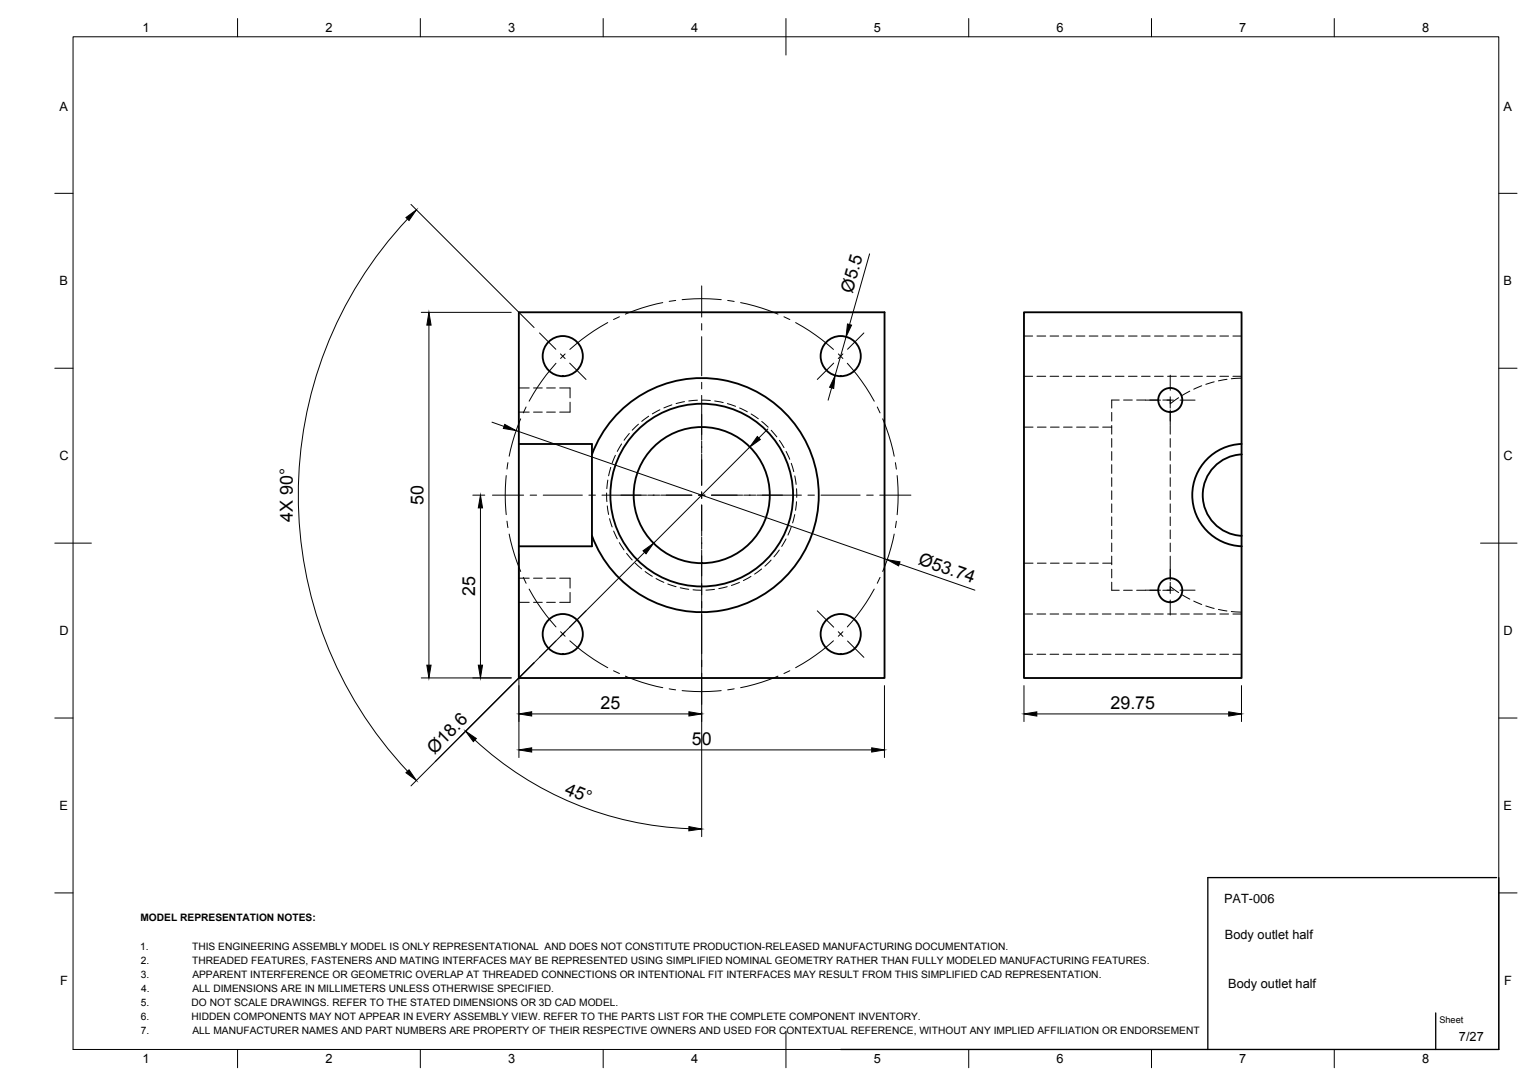
ISO-10303-21;
HEADER;
/* Generated by software containing ST-Developer
 * from STEP Tools, Inc. (www.steptools.com) 
 */

FILE_DESCRIPTION(
/* description */ ('Ball-type isolation valve (generic)'),
/* implementation_level */ '2;1');

FILE_NAME(
/* name */ 'Body outlet half.step',
/* time_stamp */ '2026-10-27T10:53:05-07:00',
/* author */ (''),
/* organization */ (''),
/* preprocessor_version */ 'ST-DEVELOPER v20.2',
/* originating_system */ 'Autodesk Translation Framework v15.17.0.0',
/* authorisation */ '');

FILE_SCHEMA (('AUTOMOTIVE_DESIGN { 1 0 10303 214 3 1 1 }'));
ENDSEC;

DATA;
#10=MECHANICAL_DESIGN_GEOMETRIC_PRESENTATION_REPRESENTATION('',(#279),#7425);
#227=SHAPE_REPRESENTATION_RELATIONSHIP('SRR','None',#7537,#253);
#253=ADVANCED_BREP_SHAPE_REPRESENTATION('',(#305),#7400);
#279=STYLED_ITEM('',(#7723),#305);
#305=MANIFOLD_SOLID_BREP('Body1',#4084);
#328=SPHERICAL_SURFACE('',#4490,1.6);
#348=FACE_BOUND('',#882,.T.);
#349=FACE_BOUND('',#883,.T.);
#350=FACE_BOUND('',#887,.T.);
#351=FACE_BOUND('',#889,.T.);
#352=FACE_BOUND('',#891,.T.);
#353=FACE_BOUND('',#893,.T.);
#354=FACE_BOUND('',#894,.T.);
#355=FACE_BOUND('',#895,.T.);
#356=FACE_BOUND('',#896,.T.);
#357=FACE_BOUND('',#897,.T.);
#358=FACE_BOUND('',#900,.T.);
#359=FACE_BOUND('',#901,.T.);
#360=FACE_BOUND('',#902,.T.);
#361=FACE_BOUND('',#903,.T.);
#432=PLANE('',#4458);
#433=PLANE('',#4462);
#434=PLANE('',#4478);
#435=PLANE('',#4480);
#436=PLANE('',#4487);
#437=PLANE('',#4488);
#438=PLANE('',#4492);
#439=PLANE('',#4493);
#440=PLANE('',#4494);
#441=PLANE('',#4495);
#442=PLANE('',#4496);
#605=FACE_OUTER_BOUND('',#871,.T.);
#606=FACE_OUTER_BOUND('',#872,.T.);
#607=FACE_OUTER_BOUND('',#873,.T.);
#608=FACE_OUTER_BOUND('',#874,.T.);
#609=FACE_OUTER_BOUND('',#875,.T.);
#610=FACE_OUTER_BOUND('',#876,.T.);
#611=FACE_OUTER_BOUND('',#877,.T.);
#612=FACE_OUTER_BOUND('',#878,.T.);
#613=FACE_OUTER_BOUND('',#879,.T.);
#614=FACE_OUTER_BOUND('',#880,.T.);
#615=FACE_OUTER_BOUND('',#881,.T.);
#616=FACE_OUTER_BOUND('',#884,.T.);
#617=FACE_OUTER_BOUND('',#885,.T.);
#618=FACE_OUTER_BOUND('',#886,.T.);
#619=FACE_OUTER_BOUND('',#888,.T.);
#620=FACE_OUTER_BOUND('',#890,.T.);
#621=FACE_OUTER_BOUND('',#892,.T.);
#622=FACE_OUTER_BOUND('',#898,.T.);
#623=FACE_OUTER_BOUND('',#899,.T.);
#624=FACE_OUTER_BOUND('',#904,.T.);
#625=FACE_OUTER_BOUND('',#905,.T.);
#871=EDGE_LOOP('',(#2881,#2882,#2883,#2884));
#872=EDGE_LOOP('',(#2885));
#873=EDGE_LOOP('',(#2886,#2887,#2888,#2889));
#874=EDGE_LOOP('',(#2890));
#875=EDGE_LOOP('',(#2891,#2892,#2893,#2894));
#876=EDGE_LOOP('',(#2895,#2896,#2897,#2898));
#877=EDGE_LOOP('',(#2899,#2900,#2901,#2902));
#878=EDGE_LOOP('',(#2903,#2904,#2905,#2906));
#879=EDGE_LOOP('',(#2907,#2908,#2909,#2910));
#880=EDGE_LOOP('',(#2911,#2912,#2913,#2914));
#881=EDGE_LOOP('',(#2915,#2916,#2917,#2918,#2919,#2920));
#882=EDGE_LOOP('',(#2921));
#883=EDGE_LOOP('',(#2922));
#884=EDGE_LOOP('',(#2923,#2924,#2925,#2926));
#885=EDGE_LOOP('',(#2927,#2928,#2929,#2930));
#886=EDGE_LOOP('',(#2931));
#887=EDGE_LOOP('',(#2932));
#888=EDGE_LOOP('',(#2933));
#889=EDGE_LOOP('',(#2934));
#890=EDGE_LOOP('',(#2935,#2936));
#891=EDGE_LOOP('',(#2937));
#892=EDGE_LOOP('',(#2938,#2939,#2940,#2941));
#893=EDGE_LOOP('',(#2942));
#894=EDGE_LOOP('',(#2943));
#895=EDGE_LOOP('',(#2944));
#896=EDGE_LOOP('',(#2945));
#897=EDGE_LOOP('',(#2946));
#898=EDGE_LOOP('',(#2947,#2948,#2949,#2950));
#899=EDGE_LOOP('',(#2951,#2952,#2953,#2954,#2955,#2956,#2957,#2958,#2959,
#2960));
#900=EDGE_LOOP('',(#2961));
#901=EDGE_LOOP('',(#2962));
#902=EDGE_LOOP('',(#2963));
#903=EDGE_LOOP('',(#2964));
#904=EDGE_LOOP('',(#2965,#2966,#2967,#2968));
#905=EDGE_LOOP('',(#2969,#2970,#2971,#2972));
#1192=LINE('',#6324,#1500);
#1193=LINE('',#6331,#1501);
#1194=LINE('',#6338,#1502);
#1195=LINE('',#6344,#1503);
#1196=LINE('',#6350,#1504);
#1197=LINE('',#6356,#1505);
#1198=LINE('',#6361,#1506);
#1199=LINE('',#6365,#1507);
#1200=LINE('',#6369,#1508);
#1201=LINE('',#6372,#1509);
#1202=LINE('',#6375,#1510);
#1203=LINE('',#6377,#1511);
#1204=LINE('',#6379,#1512);
#1205=LINE('',#6381,#1513);
#1206=LINE('',#6382,#1514);
#1207=LINE('',#6387,#1515);
#1208=LINE('',#6393,#1516);
#1209=LINE('',#6404,#1517);
#1210=LINE('',#6405,#1518);
#1211=LINE('',#6406,#1519);
#1212=LINE('',#6409,#1520);
#1213=LINE('',#6410,#1521);
#1214=LINE('',#6413,#1522);
#1215=LINE('',#6414,#1523);
#1216=LINE('',#6416,#1524);
#1500=VECTOR('',#5041,0.165);
#1501=VECTOR('',#5050,0.165);
#1502=VECTOR('',#5059,0.275);
#1503=VECTOR('',#5066,0.275);
#1504=VECTOR('',#5073,0.275);
#1505=VECTOR('',#5080,0.275);
#1506=VECTOR('',#5085,1.);
#1507=VECTOR('',#5088,1.);
#1508=VECTOR('',#5093,1.);
#1509=VECTOR('',#5096,1.);
#1510=VECTOR('',#5099,1.);
#1511=VECTOR('',#5100,1.);
#1512=VECTOR('',#5101,1.);
#1513=VECTOR('',#5102,1.);
#1514=VECTOR('',#5103,1.);
#1515=VECTOR('',#5108,0.93);
#1516=VECTOR('',#5115,1.3);
#1517=VECTOR('',#5130,1.);
#1518=VECTOR('',#5131,1.);
#1519=VECTOR('',#5132,1.);
#1520=VECTOR('',#5135,1.);
#1521=VECTOR('',#5136,1.);
#1522=VECTOR('',#5139,1.);
#1523=VECTOR('',#5140,1.);
#1524=VECTOR('',#5143,1.);
#1807=CIRCLE('',#4456,0.165);
#1808=CIRCLE('',#4457,0.165);
#1809=CIRCLE('',#4460,0.165);
#1810=CIRCLE('',#4461,0.165);
#1811=CIRCLE('',#4464,0.275);
#1812=CIRCLE('',#4465,0.275);
#1813=CIRCLE('',#4467,0.275);
#1814=CIRCLE('',#4468,0.275);
#1815=CIRCLE('',#4470,0.275);
#1816=CIRCLE('',#4471,0.275);
#1817=CIRCLE('',#4473,0.275);
#1818=CIRCLE('',#4474,0.275);
#1819=CIRCLE('',#4476,0.7);
#1820=CIRCLE('',#4477,0.7);
#1821=CIRCLE('',#4479,0.556776436283003);
#1822=CIRCLE('',#4482,0.93);
#1823=CIRCLE('',#4483,0.93);
#1824=CIRCLE('',#4485,1.3);
#1825=CIRCLE('',#4486,1.3);
#1826=CIRCLE('',#4489,1.24899959967968);
#1827=CIRCLE('',#4491,1.59980467557762);
#1992=VERTEX_POINT('',#6321);
#1993=VERTEX_POINT('',#6323);
#1994=VERTEX_POINT('',#6328);
#1995=VERTEX_POINT('',#6330);
#1996=VERTEX_POINT('',#6335);
#1997=VERTEX_POINT('',#6337);
#1998=VERTEX_POINT('',#6341);
#1999=VERTEX_POINT('',#6343);
#2000=VERTEX_POINT('',#6347);
#2001=VERTEX_POINT('',#6349);
#2002=VERTEX_POINT('',#6353);
#2003=VERTEX_POINT('',#6355);
#2004=VERTEX_POINT('',#6359);
#2005=VERTEX_POINT('',#6360);
#2006=VERTEX_POINT('',#6362);
#2007=VERTEX_POINT('',#6364);
#2008=VERTEX_POINT('',#6368);
#2009=VERTEX_POINT('',#6370);
#2010=VERTEX_POINT('',#6374);
#2011=VERTEX_POINT('',#6376);
#2012=VERTEX_POINT('',#6378);
#2013=VERTEX_POINT('',#6380);
#2014=VERTEX_POINT('',#6384);
#2015=VERTEX_POINT('',#6386);
#2016=VERTEX_POINT('',#6390);
#2017=VERTEX_POINT('',#6392);
#2018=VERTEX_POINT('',#6397);
#2019=VERTEX_POINT('',#6402);
#2020=VERTEX_POINT('',#6403);
#2021=VERTEX_POINT('',#6408);
#2022=VERTEX_POINT('',#6412);
#2333=EDGE_CURVE('',#1992,#1992,#1807,.T.);
#2334=EDGE_CURVE('',#1992,#1993,#1192,.T.);
#2335=EDGE_CURVE('',#1993,#1993,#1808,.T.);
#2336=EDGE_CURVE('',#1994,#1994,#1809,.T.);
#2337=EDGE_CURVE('',#1994,#1995,#1193,.T.);
#2338=EDGE_CURVE('',#1995,#1995,#1810,.T.);
#2339=EDGE_CURVE('',#1996,#1996,#1811,.T.);
#2340=EDGE_CURVE('',#1996,#1997,#1194,.T.);
#2341=EDGE_CURVE('',#1997,#1997,#1812,.T.);
#2342=EDGE_CURVE('',#1998,#1998,#1813,.T.);
#2343=EDGE_CURVE('',#1998,#1999,#1195,.T.);
#2344=EDGE_CURVE('',#1999,#1999,#1814,.T.);
#2345=EDGE_CURVE('',#2000,#2000,#1815,.T.);
#2346=EDGE_CURVE('',#2000,#2001,#1196,.T.);
#2347=EDGE_CURVE('',#2001,#2001,#1816,.T.);
#2348=EDGE_CURVE('',#2002,#2002,#1817,.T.);
#2349=EDGE_CURVE('',#2002,#2003,#1197,.T.);
#2350=EDGE_CURVE('',#2003,#2003,#1818,.T.);
#2351=EDGE_CURVE('',#2004,#2005,#1198,.T.);
#2352=EDGE_CURVE('',#2006,#2004,#1819,.T.);
#2353=EDGE_CURVE('',#2007,#2006,#1199,.T.);
#2354=EDGE_CURVE('',#2005,#2007,#1820,.T.);
#2355=EDGE_CURVE('',#2008,#2004,#1200,.T.);
#2356=EDGE_CURVE('',#2009,#2008,#1821,.T.);
#2357=EDGE_CURVE('',#2006,#2009,#1201,.T.);
#2358=EDGE_CURVE('',#2007,#2010,#1202,.T.);
#2359=EDGE_CURVE('',#2010,#2011,#1203,.T.);
#2360=EDGE_CURVE('',#2011,#2012,#1204,.T.);
#2361=EDGE_CURVE('',#2012,#2013,#1205,.T.);
#2362=EDGE_CURVE('',#2013,#2005,#1206,.T.);
#2363=EDGE_CURVE('',#2014,#2014,#1822,.T.);
#2364=EDGE_CURVE('',#2014,#2015,#1207,.T.);
#2365=EDGE_CURVE('',#2015,#2015,#1823,.T.);
#2366=EDGE_CURVE('',#2016,#2016,#1824,.T.);
#2367=EDGE_CURVE('',#2016,#2017,#1208,.T.);
#2368=EDGE_CURVE('',#2017,#2017,#1825,.T.);
#2369=EDGE_CURVE('',#2018,#2018,#1826,.T.);
#2370=EDGE_CURVE('',#2009,#2008,#1827,.T.);
#2371=EDGE_CURVE('',#2019,#2020,#1209,.T.);
#2372=EDGE_CURVE('',#2020,#2012,#1210,.T.);
#2373=EDGE_CURVE('',#2019,#2011,#1211,.T.);
#2374=EDGE_CURVE('',#2021,#2019,#1212,.T.);
#2375=EDGE_CURVE('',#2021,#2010,#1213,.T.);
#2376=EDGE_CURVE('',#2022,#2013,#1214,.T.);
#2377=EDGE_CURVE('',#2022,#2021,#1215,.T.);
#2378=EDGE_CURVE('',#2020,#2022,#1216,.T.);
#2881=ORIENTED_EDGE('',*,*,#2333,.F.);
#2882=ORIENTED_EDGE('',*,*,#2334,.T.);
#2883=ORIENTED_EDGE('',*,*,#2335,.F.);
#2884=ORIENTED_EDGE('',*,*,#2334,.F.);
#2885=ORIENTED_EDGE('',*,*,#2333,.T.);
#2886=ORIENTED_EDGE('',*,*,#2336,.F.);
#2887=ORIENTED_EDGE('',*,*,#2337,.T.);
#2888=ORIENTED_EDGE('',*,*,#2338,.F.);
#2889=ORIENTED_EDGE('',*,*,#2337,.F.);
#2890=ORIENTED_EDGE('',*,*,#2336,.T.);
#2891=ORIENTED_EDGE('',*,*,#2339,.F.);
#2892=ORIENTED_EDGE('',*,*,#2340,.T.);
#2893=ORIENTED_EDGE('',*,*,#2341,.F.);
#2894=ORIENTED_EDGE('',*,*,#2340,.F.);
#2895=ORIENTED_EDGE('',*,*,#2342,.F.);
#2896=ORIENTED_EDGE('',*,*,#2343,.T.);
#2897=ORIENTED_EDGE('',*,*,#2344,.F.);
#2898=ORIENTED_EDGE('',*,*,#2343,.F.);
#2899=ORIENTED_EDGE('',*,*,#2345,.F.);
#2900=ORIENTED_EDGE('',*,*,#2346,.T.);
#2901=ORIENTED_EDGE('',*,*,#2347,.F.);
#2902=ORIENTED_EDGE('',*,*,#2346,.F.);
#2903=ORIENTED_EDGE('',*,*,#2348,.F.);
#2904=ORIENTED_EDGE('',*,*,#2349,.T.);
#2905=ORIENTED_EDGE('',*,*,#2350,.F.);
#2906=ORIENTED_EDGE('',*,*,#2349,.F.);
#2907=ORIENTED_EDGE('',*,*,#2351,.F.);
#2908=ORIENTED_EDGE('',*,*,#2352,.F.);
#2909=ORIENTED_EDGE('',*,*,#2353,.F.);
#2910=ORIENTED_EDGE('',*,*,#2354,.F.);
#2911=ORIENTED_EDGE('',*,*,#2355,.F.);
#2912=ORIENTED_EDGE('',*,*,#2356,.F.);
#2913=ORIENTED_EDGE('',*,*,#2357,.F.);
#2914=ORIENTED_EDGE('',*,*,#2352,.T.);
#2915=ORIENTED_EDGE('',*,*,#2354,.T.);
#2916=ORIENTED_EDGE('',*,*,#2358,.T.);
#2917=ORIENTED_EDGE('',*,*,#2359,.T.);
#2918=ORIENTED_EDGE('',*,*,#2360,.T.);
#2919=ORIENTED_EDGE('',*,*,#2361,.T.);
#2920=ORIENTED_EDGE('',*,*,#2362,.T.);
#2921=ORIENTED_EDGE('',*,*,#2335,.T.);
#2922=ORIENTED_EDGE('',*,*,#2338,.T.);
#2923=ORIENTED_EDGE('',*,*,#2363,.F.);
#2924=ORIENTED_EDGE('',*,*,#2364,.T.);
#2925=ORIENTED_EDGE('',*,*,#2365,.F.);
#2926=ORIENTED_EDGE('',*,*,#2364,.F.);
#2927=ORIENTED_EDGE('',*,*,#2366,.F.);
#2928=ORIENTED_EDGE('',*,*,#2367,.T.);
#2929=ORIENTED_EDGE('',*,*,#2368,.T.);
#2930=ORIENTED_EDGE('',*,*,#2367,.F.);
#2931=ORIENTED_EDGE('',*,*,#2368,.F.);
#2932=ORIENTED_EDGE('',*,*,#2363,.T.);
#2933=ORIENTED_EDGE('',*,*,#2366,.T.);
#2934=ORIENTED_EDGE('',*,*,#2369,.F.);
#2935=ORIENTED_EDGE('',*,*,#2356,.T.);
#2936=ORIENTED_EDGE('',*,*,#2370,.F.);
#2937=ORIENTED_EDGE('',*,*,#2369,.T.);
#2938=ORIENTED_EDGE('',*,*,#2371,.T.);
#2939=ORIENTED_EDGE('',*,*,#2372,.T.);
#2940=ORIENTED_EDGE('',*,*,#2360,.F.);
#2941=ORIENTED_EDGE('',*,*,#2373,.F.);
#2942=ORIENTED_EDGE('',*,*,#2365,.T.);
#2943=ORIENTED_EDGE('',*,*,#2350,.T.);
#2944=ORIENTED_EDGE('',*,*,#2347,.T.);
#2945=ORIENTED_EDGE('',*,*,#2344,.T.);
#2946=ORIENTED_EDGE('',*,*,#2341,.T.);
#2947=ORIENTED_EDGE('',*,*,#2374,.T.);
#2948=ORIENTED_EDGE('',*,*,#2373,.T.);
#2949=ORIENTED_EDGE('',*,*,#2359,.F.);
#2950=ORIENTED_EDGE('',*,*,#2375,.F.);
#2951=ORIENTED_EDGE('',*,*,#2351,.T.);
#2952=ORIENTED_EDGE('',*,*,#2362,.F.);
#2953=ORIENTED_EDGE('',*,*,#2376,.F.);
#2954=ORIENTED_EDGE('',*,*,#2377,.T.);
#2955=ORIENTED_EDGE('',*,*,#2375,.T.);
#2956=ORIENTED_EDGE('',*,*,#2358,.F.);
#2957=ORIENTED_EDGE('',*,*,#2353,.T.);
#2958=ORIENTED_EDGE('',*,*,#2357,.T.);
#2959=ORIENTED_EDGE('',*,*,#2370,.T.);
#2960=ORIENTED_EDGE('',*,*,#2355,.T.);
#2961=ORIENTED_EDGE('',*,*,#2339,.T.);
#2962=ORIENTED_EDGE('',*,*,#2342,.T.);
#2963=ORIENTED_EDGE('',*,*,#2345,.T.);
#2964=ORIENTED_EDGE('',*,*,#2348,.T.);
#2965=ORIENTED_EDGE('',*,*,#2378,.T.);
#2966=ORIENTED_EDGE('',*,*,#2376,.T.);
#2967=ORIENTED_EDGE('',*,*,#2361,.F.);
#2968=ORIENTED_EDGE('',*,*,#2372,.F.);
#2969=ORIENTED_EDGE('',*,*,#2378,.F.);
#2970=ORIENTED_EDGE('',*,*,#2371,.F.);
#2971=ORIENTED_EDGE('',*,*,#2374,.F.);
#2972=ORIENTED_EDGE('',*,*,#2377,.F.);
#3776=CYLINDRICAL_SURFACE('',#4455,0.165);
#3777=CYLINDRICAL_SURFACE('',#4459,0.165);
#3778=CYLINDRICAL_SURFACE('',#4463,0.275);
#3779=CYLINDRICAL_SURFACE('',#4466,0.275);
#3780=CYLINDRICAL_SURFACE('',#4469,0.275);
#3781=CYLINDRICAL_SURFACE('',#4472,0.275);
#3782=CYLINDRICAL_SURFACE('',#4475,0.7);
#3783=CYLINDRICAL_SURFACE('',#4481,0.93);
#3784=CYLINDRICAL_SURFACE('',#4484,1.3);
#3859=ADVANCED_FACE('',(#605),#3776,.F.);
#3860=ADVANCED_FACE('',(#606),#432,.T.);
#3861=ADVANCED_FACE('',(#607),#3777,.F.);
#3862=ADVANCED_FACE('',(#608),#433,.T.);
#3863=ADVANCED_FACE('',(#609),#3778,.F.);
#3864=ADVANCED_FACE('',(#610),#3779,.F.);
#3865=ADVANCED_FACE('',(#611),#3780,.F.);
#3866=ADVANCED_FACE('',(#612),#3781,.F.);
#3867=ADVANCED_FACE('',(#613),#3782,.F.);
#3868=ADVANCED_FACE('',(#614),#434,.T.);
#3869=ADVANCED_FACE('',(#615,#348,#349),#435,.T.);
#3870=ADVANCED_FACE('',(#616),#3783,.F.);
#3871=ADVANCED_FACE('',(#617),#3784,.F.);
#3872=ADVANCED_FACE('',(#618,#350),#436,.F.);
#3873=ADVANCED_FACE('',(#619,#351),#437,.T.);
#3874=ADVANCED_FACE('',(#620,#352),#328,.F.);
#3875=ADVANCED_FACE('',(#621,#353,#354,#355,#356,#357),#438,.T.);
#3876=ADVANCED_FACE('',(#622),#439,.T.);
#3877=ADVANCED_FACE('',(#623,#358,#359,#360,#361),#440,.T.);
#3878=ADVANCED_FACE('',(#624),#441,.T.);
#3879=ADVANCED_FACE('',(#625),#442,.F.);
#4084=CLOSED_SHELL('',(#3859,#3860,#3861,#3862,#3863,#3864,#3865,#3866,
#3867,#3868,#3869,#3870,#3871,#3872,#3873,#3874,#3875,#3876,#3877,#3878,
#3879));
#4454=AXIS2_PLACEMENT_3D('',#6319,#5035,#5036);
#4455=AXIS2_PLACEMENT_3D('',#6320,#5037,#5038);
#4456=AXIS2_PLACEMENT_3D('',#6322,#5039,#5040);
#4457=AXIS2_PLACEMENT_3D('',#6325,#5042,#5043);
#4458=AXIS2_PLACEMENT_3D('',#6326,#5044,#5045);
#4459=AXIS2_PLACEMENT_3D('',#6327,#5046,#5047);
#4460=AXIS2_PLACEMENT_3D('',#6329,#5048,#5049);
#4461=AXIS2_PLACEMENT_3D('',#6332,#5051,#5052);
#4462=AXIS2_PLACEMENT_3D('',#6333,#5053,#5054);
#4463=AXIS2_PLACEMENT_3D('',#6334,#5055,#5056);
#4464=AXIS2_PLACEMENT_3D('',#6336,#5057,#5058);
#4465=AXIS2_PLACEMENT_3D('',#6339,#5060,#5061);
#4466=AXIS2_PLACEMENT_3D('',#6340,#5062,#5063);
#4467=AXIS2_PLACEMENT_3D('',#6342,#5064,#5065);
#4468=AXIS2_PLACEMENT_3D('',#6345,#5067,#5068);
#4469=AXIS2_PLACEMENT_3D('',#6346,#5069,#5070);
#4470=AXIS2_PLACEMENT_3D('',#6348,#5071,#5072);
#4471=AXIS2_PLACEMENT_3D('',#6351,#5074,#5075);
#4472=AXIS2_PLACEMENT_3D('',#6352,#5076,#5077);
#4473=AXIS2_PLACEMENT_3D('',#6354,#5078,#5079);
#4474=AXIS2_PLACEMENT_3D('',#6357,#5081,#5082);
#4475=AXIS2_PLACEMENT_3D('',#6358,#5083,#5084);
#4476=AXIS2_PLACEMENT_3D('',#6363,#5086,#5087);
#4477=AXIS2_PLACEMENT_3D('',#6366,#5089,#5090);
#4478=AXIS2_PLACEMENT_3D('',#6367,#5091,#5092);
#4479=AXIS2_PLACEMENT_3D('',#6371,#5094,#5095);
#4480=AXIS2_PLACEMENT_3D('',#6373,#5097,#5098);
#4481=AXIS2_PLACEMENT_3D('',#6383,#5104,#5105);
#4482=AXIS2_PLACEMENT_3D('',#6385,#5106,#5107);
#4483=AXIS2_PLACEMENT_3D('',#6388,#5109,#5110);
#4484=AXIS2_PLACEMENT_3D('',#6389,#5111,#5112);
#4485=AXIS2_PLACEMENT_3D('',#6391,#5113,#5114);
#4486=AXIS2_PLACEMENT_3D('',#6394,#5116,#5117);
#4487=AXIS2_PLACEMENT_3D('',#6395,#5118,#5119);
#4488=AXIS2_PLACEMENT_3D('',#6396,#5120,#5121);
#4489=AXIS2_PLACEMENT_3D('',#6398,#5122,#5123);
#4490=AXIS2_PLACEMENT_3D('',#6399,#5124,#5125);
#4491=AXIS2_PLACEMENT_3D('',#6400,#5126,#5127);
#4492=AXIS2_PLACEMENT_3D('',#6401,#5128,#5129);
#4493=AXIS2_PLACEMENT_3D('',#6407,#5133,#5134);
#4494=AXIS2_PLACEMENT_3D('',#6411,#5137,#5138);
#4495=AXIS2_PLACEMENT_3D('',#6415,#5141,#5142);
#4496=AXIS2_PLACEMENT_3D('',#6417,#5144,#5145);
#5035=DIRECTION('axis',(0.,0.,1.));
#5036=DIRECTION('refdir',(1.,0.,0.));
#5037=DIRECTION('center_axis',(0.,0.,1.));
#5038=DIRECTION('ref_axis',(1.,0.,0.));
#5039=DIRECTION('center_axis',(0.,0.,1.));
#5040=DIRECTION('ref_axis',(1.,0.,0.));
#5041=DIRECTION('',(0.,0.,1.));
#5042=DIRECTION('center_axis',(0.,0.,-1.));
#5043=DIRECTION('ref_axis',(1.,0.,0.));
#5044=DIRECTION('center_axis',(0.,0.,1.));
#5045=DIRECTION('ref_axis',(1.,0.,0.));
#5046=DIRECTION('center_axis',(0.,0.,1.));
#5047=DIRECTION('ref_axis',(1.,0.,0.));
#5048=DIRECTION('center_axis',(0.,0.,1.));
#5049=DIRECTION('ref_axis',(1.,0.,0.));
#5050=DIRECTION('',(0.,0.,1.));
#5051=DIRECTION('center_axis',(0.,0.,-1.));
#5052=DIRECTION('ref_axis',(1.,0.,0.));
#5053=DIRECTION('center_axis',(0.,0.,1.));
#5054=DIRECTION('ref_axis',(1.,0.,0.));
#5055=DIRECTION('center_axis',(0.,1.,0.));
#5056=DIRECTION('ref_axis',(1.,0.,0.));
#5057=DIRECTION('center_axis',(0.,1.,0.));
#5058=DIRECTION('ref_axis',(1.,0.,0.));
#5059=DIRECTION('',(0.,1.,0.));
#5060=DIRECTION('center_axis',(0.,-1.,0.));
#5061=DIRECTION('ref_axis',(1.,0.,0.));
#5062=DIRECTION('center_axis',(0.,1.,0.));
#5063=DIRECTION('ref_axis',(1.,0.,0.));
#5064=DIRECTION('center_axis',(0.,1.,0.));
#5065=DIRECTION('ref_axis',(1.,0.,0.));
#5066=DIRECTION('',(0.,1.,0.));
#5067=DIRECTION('center_axis',(0.,-1.,0.));
#5068=DIRECTION('ref_axis',(1.,0.,0.));
#5069=DIRECTION('center_axis',(0.,1.,0.));
#5070=DIRECTION('ref_axis',(1.,0.,0.));
#5071=DIRECTION('center_axis',(0.,1.,0.));
#5072=DIRECTION('ref_axis',(1.,0.,0.));
#5073=DIRECTION('',(0.,1.,0.));
#5074=DIRECTION('center_axis',(0.,-1.,0.));
#5075=DIRECTION('ref_axis',(1.,0.,0.));
#5076=DIRECTION('center_axis',(0.,1.,0.));
#5077=DIRECTION('ref_axis',(1.,0.,0.));
#5078=DIRECTION('center_axis',(0.,1.,0.));
#5079=DIRECTION('ref_axis',(1.,0.,0.));
#5080=DIRECTION('',(0.,1.,0.));
#5081=DIRECTION('center_axis',(0.,-1.,0.));
#5082=DIRECTION('ref_axis',(1.,0.,0.));
#5083=DIRECTION('center_axis',(0.,0.,1.));
#5084=DIRECTION('ref_axis',(1.,0.,0.));
#5085=DIRECTION('',(0.,0.,1.));
#5086=DIRECTION('center_axis',(0.,0.,1.));
#5087=DIRECTION('ref_axis',(1.,0.,0.));
#5088=DIRECTION('',(0.,0.,-1.));
#5089=DIRECTION('center_axis',(0.,0.,-1.));
#5090=DIRECTION('ref_axis',(1.,0.,0.));
#5091=DIRECTION('center_axis',(0.,0.,1.));
#5092=DIRECTION('ref_axis',(1.,0.,0.));
#5093=DIRECTION('',(-1.,0.,0.));
#5094=DIRECTION('center_axis',(0.,0.,1.));
#5095=DIRECTION('ref_axis',(0.,-1.,0.));
#5096=DIRECTION('',(-1.,0.,0.));
#5097=DIRECTION('center_axis',(0.,0.,1.));
#5098=DIRECTION('ref_axis',(1.,0.,0.));
#5099=DIRECTION('',(1.,0.,0.));
#5100=DIRECTION('',(0.,1.,0.));
#5101=DIRECTION('',(-1.,0.,0.));
#5102=DIRECTION('',(0.,-1.,0.));
#5103=DIRECTION('',(1.,0.,0.));
#5104=DIRECTION('center_axis',(0.,1.,0.));
#5105=DIRECTION('ref_axis',(1.,0.,0.));
#5106=DIRECTION('center_axis',(0.,1.,0.));
#5107=DIRECTION('ref_axis',(1.,0.,0.));
#5108=DIRECTION('',(0.,1.,0.));
#5109=DIRECTION('center_axis',(0.,-1.,0.));
#5110=DIRECTION('ref_axis',(1.,0.,0.));
#5111=DIRECTION('center_axis',(0.,1.,0.));
#5112=DIRECTION('ref_axis',(1.,0.,0.));
#5113=DIRECTION('center_axis',(0.,1.,0.));
#5114=DIRECTION('ref_axis',(1.,0.,0.));
#5115=DIRECTION('',(0.,1.,0.));
#5116=DIRECTION('center_axis',(0.,1.,0.));
#5117=DIRECTION('ref_axis',(1.,0.,0.));
#5118=DIRECTION('center_axis',(0.,1.,0.));
#5119=DIRECTION('ref_axis',(1.,0.,0.));
#5120=DIRECTION('center_axis',(0.,1.,0.));
#5121=DIRECTION('ref_axis',(1.,0.,0.));
#5122=DIRECTION('center_axis',(0.,1.,0.));
#5123=DIRECTION('ref_axis',(0.,0.,1.));
#5124=DIRECTION('center_axis',(6.12323399573677E-17,0.,1.));
#5125=DIRECTION('ref_axis',(1.,0.,0.));
#5126=DIRECTION('center_axis',(0.,1.,0.));
#5127=DIRECTION('ref_axis',(0.,0.,1.));
#5128=DIRECTION('center_axis',(0.,1.,0.));
#5129=DIRECTION('ref_axis',(-1.,0.,0.));
#5130=DIRECTION('',(-1.,0.,0.));
#5131=DIRECTION('',(0.,0.,1.));
#5132=DIRECTION('',(0.,0.,1.));
#5133=DIRECTION('center_axis',(1.,0.,0.));
#5134=DIRECTION('ref_axis',(0.,1.,0.));
#5135=DIRECTION('',(0.,1.,0.));
#5136=DIRECTION('',(0.,0.,1.));
#5137=DIRECTION('center_axis',(0.,-1.,0.));
#5138=DIRECTION('ref_axis',(1.,0.,0.));
#5139=DIRECTION('',(0.,0.,1.));
#5140=DIRECTION('',(1.,0.,0.));
#5141=DIRECTION('center_axis',(-1.,0.,0.));
#5142=DIRECTION('ref_axis',(0.,-1.,0.));
#5143=DIRECTION('',(0.,-1.,0.));
#5144=DIRECTION('center_axis',(0.,0.,1.));
#5145=DIRECTION('ref_axis',(1.,0.,0.));
#6319=CARTESIAN_POINT('',(0.,0.,0.));
#6320=CARTESIAN_POINT('Origin',(-1.3,1.,6.8));
#6321=CARTESIAN_POINT('',(-1.465,1.,6.8));
#6322=CARTESIAN_POINT('Origin',(-1.3,1.,6.8));
#6323=CARTESIAN_POINT('',(-1.465,1.,7.5));
#6324=CARTESIAN_POINT('',(-1.465,1.,6.8));
#6325=CARTESIAN_POINT('Origin',(-1.3,1.,7.5));
#6326=CARTESIAN_POINT('Origin',(-1.3,1.,6.8));
#6327=CARTESIAN_POINT('Origin',(1.3,1.,6.8));
#6328=CARTESIAN_POINT('',(1.135,1.,6.8));
#6329=CARTESIAN_POINT('Origin',(1.3,1.,6.8));
#6330=CARTESIAN_POINT('',(1.135,1.,7.5));
#6331=CARTESIAN_POINT('',(1.135,1.,6.8));
#6332=CARTESIAN_POINT('Origin',(1.3,1.,7.5));
#6333=CARTESIAN_POINT('Origin',(1.3,1.,6.8));
#6334=CARTESIAN_POINT('Origin',(1.9,-3.1,3.1));
#6335=CARTESIAN_POINT('',(1.625,0.0249999999999999,3.1));
#6336=CARTESIAN_POINT('Origin',(1.9,0.0249999999999999,3.1));
#6337=CARTESIAN_POINT('',(1.625,3.,3.1));
#6338=CARTESIAN_POINT('',(1.625,-3.1,3.1));
#6339=CARTESIAN_POINT('Origin',(1.9,3.,3.1));
#6340=CARTESIAN_POINT('Origin',(-1.9,-3.1,6.9));
#6341=CARTESIAN_POINT('',(-2.175,0.0249999999999999,6.9));
#6342=CARTESIAN_POINT('Origin',(-1.9,0.0249999999999999,6.9));
#6343=CARTESIAN_POINT('',(-2.175,3.,6.9));
#6344=CARTESIAN_POINT('',(-2.175,-3.1,6.9));
#6345=CARTESIAN_POINT('Origin',(-1.9,3.,6.9));
#6346=CARTESIAN_POINT('Origin',(-1.9,-3.1,3.1));
#6347=CARTESIAN_POINT('',(-2.175,0.0249999999999999,3.1));
#6348=CARTESIAN_POINT('Origin',(-1.9,0.0249999999999999,3.1));
#6349=CARTESIAN_POINT('',(-2.175,3.,3.1));
#6350=CARTESIAN_POINT('',(-2.175,-3.1,3.1));
#6351=CARTESIAN_POINT('Origin',(-1.9,3.,3.1));
#6352=CARTESIAN_POINT('Origin',(1.9,-3.1,6.9));
#6353=CARTESIAN_POINT('',(1.625,0.0249999999999999,6.9));
#6354=CARTESIAN_POINT('Origin',(1.9,0.0249999999999999,6.9));
#6355=CARTESIAN_POINT('',(1.625,3.,6.9));
#6356=CARTESIAN_POINT('',(1.625,-3.1,6.9));
#6357=CARTESIAN_POINT('Origin',(1.9,3.,6.9));
#6358=CARTESIAN_POINT('Origin',(0.,0.,6.5));
#6359=CARTESIAN_POINT('',(-0.699553428981661,0.025,6.5));
#6360=CARTESIAN_POINT('',(-0.699553428981661,0.025,7.5));
#6361=CARTESIAN_POINT('',(-0.699553428981661,0.025,6.5));
#6362=CARTESIAN_POINT('',(0.699553428981661,0.025,6.5));
#6363=CARTESIAN_POINT('Origin',(0.,0.,6.5));
#6364=CARTESIAN_POINT('',(0.699553428981661,0.025,7.5));
#6365=CARTESIAN_POINT('',(0.699553428981661,0.025,6.5));
#6366=CARTESIAN_POINT('Origin',(0.,0.,7.5));
#6367=CARTESIAN_POINT('Origin',(0.,0.,6.5));
#6368=CARTESIAN_POINT('',(-0.556214886532175,0.025,6.5));
#6369=CARTESIAN_POINT('',(-1.25,0.025,6.5));
#6370=CARTESIAN_POINT('',(0.556214886532175,0.025,6.5));
#6371=CARTESIAN_POINT('Origin',(0.,0.,6.5));
#6372=CARTESIAN_POINT('',(-1.25,0.025,6.5));
#6373=CARTESIAN_POINT('Origin',(0.,1.5125,7.5));
#6374=CARTESIAN_POINT('',(2.5,0.0249999999999999,7.5));
#6375=CARTESIAN_POINT('',(-2.5,0.025,7.5));
#6376=CARTESIAN_POINT('',(2.5,3.,7.5));
#6377=CARTESIAN_POINT('',(2.5,0.025,7.5));
#6378=CARTESIAN_POINT('',(-2.5,3.,7.5));
#6379=CARTESIAN_POINT('',(2.5,3.,7.5));
#6380=CARTESIAN_POINT('',(-2.5,0.0249999999999999,7.5));
#6381=CARTESIAN_POINT('',(-2.5,3.,7.5));
#6382=CARTESIAN_POINT('',(-2.5,0.025,7.5));
#6383=CARTESIAN_POINT('Origin',(0.,1.8,5.));
#6384=CARTESIAN_POINT('',(-0.93,1.8,5.));
#6385=CARTESIAN_POINT('Origin',(0.,1.8,5.));
#6386=CARTESIAN_POINT('',(-0.93,3.,5.));
#6387=CARTESIAN_POINT('',(-0.93,1.8,5.));
#6388=CARTESIAN_POINT('Origin',(0.,3.,5.));
#6389=CARTESIAN_POINT('Origin',(0.,1.,5.));
#6390=CARTESIAN_POINT('',(-1.3,1.,5.));
#6391=CARTESIAN_POINT('Origin',(0.,1.,5.));
#6392=CARTESIAN_POINT('',(-1.3,1.8,5.));
#6393=CARTESIAN_POINT('',(-1.3,1.,5.));
#6394=CARTESIAN_POINT('Origin',(0.,1.8,5.));
#6395=CARTESIAN_POINT('Origin',(0.,1.8,5.));
#6396=CARTESIAN_POINT('Origin',(0.,1.,5.));
#6397=CARTESIAN_POINT('',(-1.52958336188405E-16,1.,3.75100040032032));
#6398=CARTESIAN_POINT('Origin',(0.,1.,5.));
#6399=CARTESIAN_POINT('Origin',(0.,0.,5.));
#6400=CARTESIAN_POINT('Origin',(0.,0.025,5.));
#6401=CARTESIAN_POINT('Origin',(2.5,3.,2.5));
#6402=CARTESIAN_POINT('',(2.5,3.,2.5));
#6403=CARTESIAN_POINT('',(-2.5,3.,2.5));
#6404=CARTESIAN_POINT('',(2.5,3.,2.5));
#6405=CARTESIAN_POINT('',(-2.5,3.,2.5));
#6406=CARTESIAN_POINT('',(2.5,3.,2.5));
#6407=CARTESIAN_POINT('Origin',(2.5,0.025,2.5));
#6408=CARTESIAN_POINT('',(2.5,0.025,2.5));
#6409=CARTESIAN_POINT('',(2.5,0.025,2.5));
#6410=CARTESIAN_POINT('',(2.5,0.025,2.5));
#6411=CARTESIAN_POINT('Origin',(-2.5,0.025,2.5));
#6412=CARTESIAN_POINT('',(-2.5,0.0249999999999999,2.5));
#6413=CARTESIAN_POINT('',(-2.5,0.0249999999999999,2.5));
#6414=CARTESIAN_POINT('',(-2.5,0.025,2.5));
#6415=CARTESIAN_POINT('Origin',(-2.5,3.,2.5));
#6416=CARTESIAN_POINT('',(-2.5,3.,2.5));
#6417=CARTESIAN_POINT('Origin',(0.,1.5125,2.5));
#7370=UNCERTAINTY_MEASURE_WITH_UNIT(LENGTH_MEASURE(0.001),#7426,
'DISTANCE_ACCURACY_VALUE',
'Maximum model space distance between geometric entities at asserted c
onnectivities');
#7395=UNCERTAINTY_MEASURE_WITH_UNIT(LENGTH_MEASURE(0.001),#7426,
'DISTANCE_ACCURACY_VALUE',
'Maximum model space distance between geometric entities at asserted c
onnectivities');
#7400=(
GEOMETRIC_REPRESENTATION_CONTEXT(3)
GLOBAL_UNCERTAINTY_ASSIGNED_CONTEXT((#7370))
GLOBAL_UNIT_ASSIGNED_CONTEXT((#7426,#7428,#7429))
REPRESENTATION_CONTEXT('','3D')
);
#7425=(
GEOMETRIC_REPRESENTATION_CONTEXT(3)
GLOBAL_UNCERTAINTY_ASSIGNED_CONTEXT((#7395))
GLOBAL_UNIT_ASSIGNED_CONTEXT((#7426,#7428,#7429))
REPRESENTATION_CONTEXT('','3D')
);
#7426=(
LENGTH_UNIT()
NAMED_UNIT(*)
SI_UNIT(.CENTI.,.METRE.)
);
#7428=(
NAMED_UNIT(*)
PLANE_ANGLE_UNIT()
SI_UNIT($,.RADIAN.)
);
#7429=(
NAMED_UNIT(*)
SI_UNIT($,.STERADIAN.)
SOLID_ANGLE_UNIT()
);
#7434=SHAPE_DEFINITION_REPRESENTATION(#7463,#7537);
#7463=PRODUCT_DEFINITION_SHAPE('',$,#7567);
#7537=SHAPE_REPRESENTATION('',(#4454),#7400);
#7562=PRODUCT_DEFINITION_CONTEXT('part definition',#7651,'design');
#7567=PRODUCT_DEFINITION('Body outlet half','Body outlet half',#7596,#7562);
#7596=PRODUCT_DEFINITION_FORMATION('',$,#7657);
#7651=APPLICATION_CONTEXT(
'Core Data for Automotive Mechanical Design Process');
#7652=PRODUCT_CONTEXT('part definition',#7651,'mechanical');
#7657=PRODUCT('Body outlet half','Body outlet half','Body outlet half',
(#7652));
#7717=COLOUR_RGB('Dark Blue',0.08,0.2,0.34);
#7718=FILL_AREA_STYLE_COLOUR('',#7717);
#7719=FILL_AREA_STYLE('',(#7718));
#7720=SURFACE_STYLE_FILL_AREA(#7719);
#7721=SURFACE_SIDE_STYLE('',(#7720));
#7722=SURFACE_STYLE_USAGE(.BOTH.,#7721);
#7723=PRESENTATION_STYLE_ASSIGNMENT((#7722));
ENDSEC;
END-ISO-10303-21;
